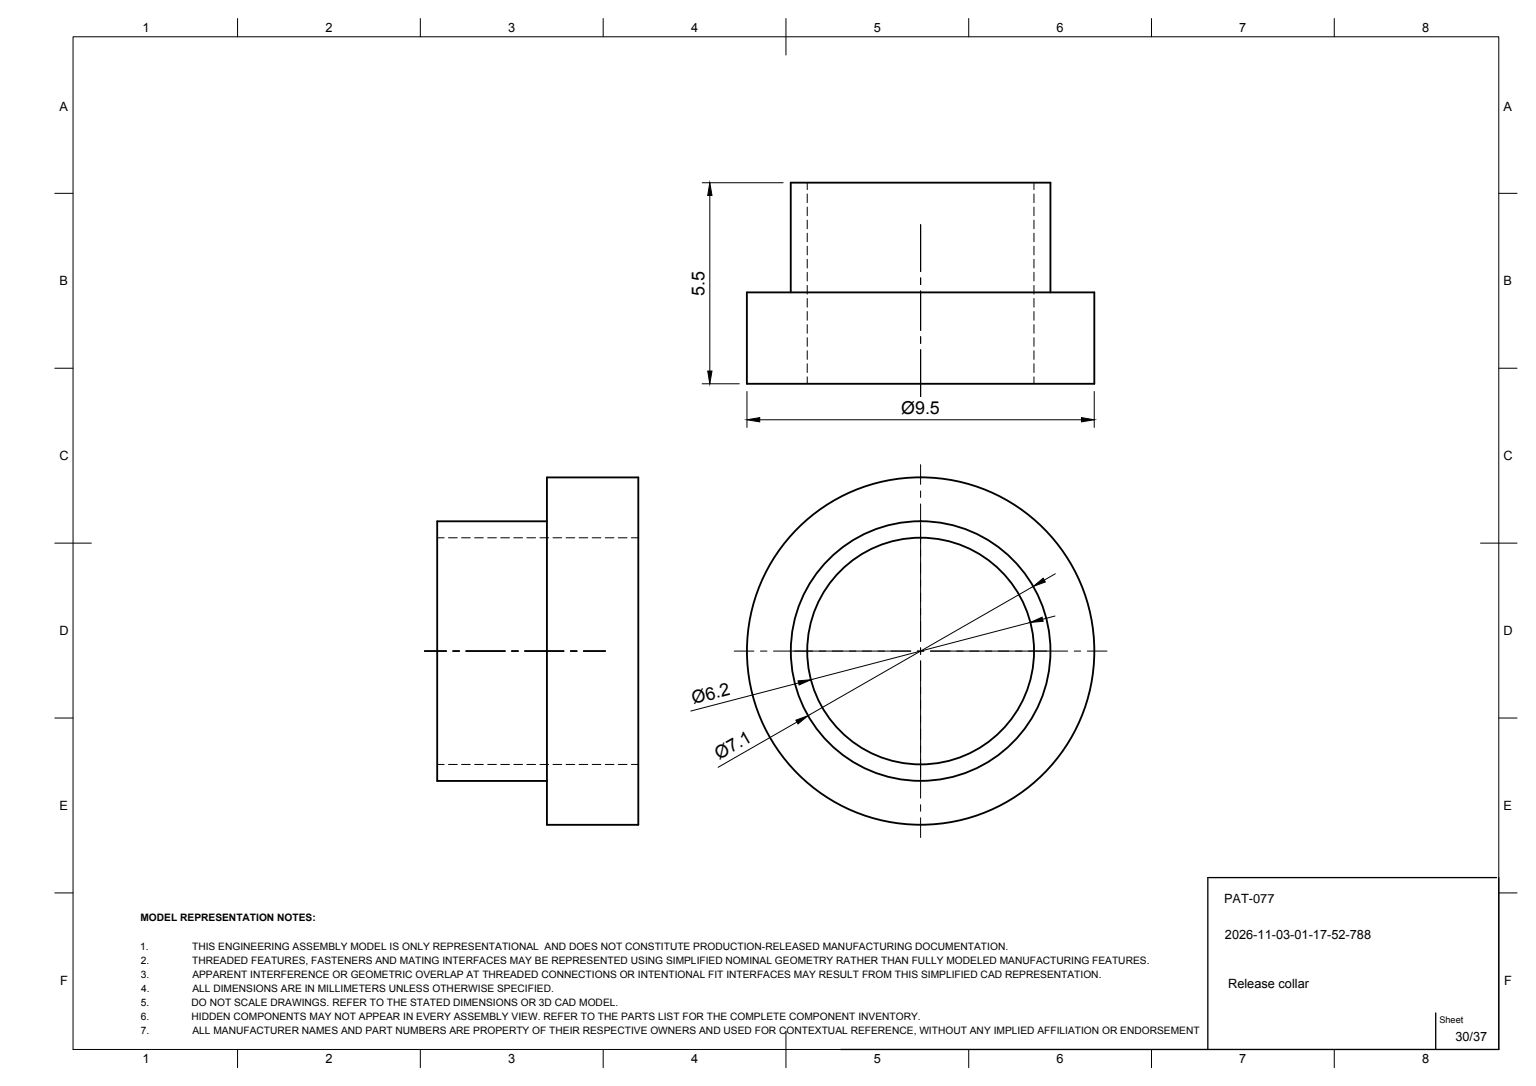
ISO-10303-21;
HEADER;
/* Generated by software containing ST-Developer
 * from STEP Tools, Inc. (www.steptools.com) 
 */

FILE_DESCRIPTION(
/* description */ ('Pallet stop with pneumatic fitting'),
/* implementation_level */ '2;1');

FILE_NAME(
/* name */ 'Release collar.step',
/* time_stamp */ '2026-10-27T10:51:41-07:00',
/* author */ (''),
/* organization */ (''),
/* preprocessor_version */ 'ST-DEVELOPER v20.2',
/* originating_system */ 'Autodesk Translation Framework v15.17.0.0',
/* authorisation */ '');

FILE_SCHEMA (('AUTOMOTIVE_DESIGN { 1 0 10303 214 3 1 1 }'));
ENDSEC;

DATA;
#10=MECHANICAL_DESIGN_GEOMETRIC_PRESENTATION_REPRESENTATION('',(#379),#10265);
#315=SHAPE_REPRESENTATION_RELATIONSHIP('SRR','None',#10430,#347);
#347=ADVANCED_BREP_SHAPE_REPRESENTATION('',(#410),#10254);
#379=STYLED_ITEM('',(#10669),#410);
#410=MANIFOLD_SOLID_BREP('Body1',#5068);
#522=FACE_BOUND('',#1371,.T.);
#523=FACE_BOUND('',#1374,.T.);
#524=FACE_BOUND('',#1377,.T.);
#672=PLANE('',#5859);
#673=PLANE('',#5864);
#674=PLANE('',#5868);
#953=FACE_OUTER_BOUND('',#1370,.T.);
#954=FACE_OUTER_BOUND('',#1372,.T.);
#955=FACE_OUTER_BOUND('',#1373,.T.);
#956=FACE_OUTER_BOUND('',#1375,.T.);
#957=FACE_OUTER_BOUND('',#1376,.T.);
#958=FACE_OUTER_BOUND('',#1378,.T.);
#1370=EDGE_LOOP('',(#4226));
#1371=EDGE_LOOP('',(#4227));
#1372=EDGE_LOOP('',(#4228,#4229,#4230,#4231));
#1373=EDGE_LOOP('',(#4232));
#1374=EDGE_LOOP('',(#4233));
#1375=EDGE_LOOP('',(#4234,#4235,#4236,#4237));
#1376=EDGE_LOOP('',(#4238));
#1377=EDGE_LOOP('',(#4239));
#1378=EDGE_LOOP('',(#4240,#4241,#4242,#4243));
#1709=LINE('',#9622,#2044);
#1710=LINE('',#9629,#2045);
#1711=LINE('',#9634,#2046);
#2044=VECTOR('',#7172,0.475);
#2045=VECTOR('',#7181,0.355);
#2046=VECTOR('',#7188,0.31);
#2342=CIRCLE('',#5860,0.475);
#2343=CIRCLE('',#5861,0.31);
#2344=CIRCLE('',#5863,0.475);
#2345=CIRCLE('',#5865,0.355);
#2346=CIRCLE('',#5867,0.355);
#2347=CIRCLE('',#5869,0.31);
#2676=VERTEX_POINT('',#9615);
#2677=VERTEX_POINT('',#9617);
#2678=VERTEX_POINT('',#9620);
#2679=VERTEX_POINT('',#9624);
#2680=VERTEX_POINT('',#9627);
#2681=VERTEX_POINT('',#9631);
#3212=EDGE_CURVE('',#2676,#2676,#2342,.T.);
#3213=EDGE_CURVE('',#2677,#2677,#2343,.T.);
#3214=EDGE_CURVE('',#2678,#2678,#2344,.T.);
#3215=EDGE_CURVE('',#2678,#2676,#1709,.T.);
#3216=EDGE_CURVE('',#2679,#2679,#2345,.T.);
#3217=EDGE_CURVE('',#2680,#2680,#2346,.T.);
#3218=EDGE_CURVE('',#2680,#2679,#1710,.T.);
#3219=EDGE_CURVE('',#2681,#2681,#2347,.T.);
#3220=EDGE_CURVE('',#2681,#2677,#1711,.T.);
#4226=ORIENTED_EDGE('',*,*,#3212,.F.);
#4227=ORIENTED_EDGE('',*,*,#3213,.T.);
#4228=ORIENTED_EDGE('',*,*,#3214,.F.);
#4229=ORIENTED_EDGE('',*,*,#3215,.T.);
#4230=ORIENTED_EDGE('',*,*,#3212,.T.);
#4231=ORIENTED_EDGE('',*,*,#3215,.F.);
#4232=ORIENTED_EDGE('',*,*,#3214,.T.);
#4233=ORIENTED_EDGE('',*,*,#3216,.F.);
#4234=ORIENTED_EDGE('',*,*,#3217,.F.);
#4235=ORIENTED_EDGE('',*,*,#3218,.T.);
#4236=ORIENTED_EDGE('',*,*,#3216,.T.);
#4237=ORIENTED_EDGE('',*,*,#3218,.F.);
#4238=ORIENTED_EDGE('',*,*,#3217,.T.);
#4239=ORIENTED_EDGE('',*,*,#3219,.F.);
#4240=ORIENTED_EDGE('',*,*,#3219,.T.);
#4241=ORIENTED_EDGE('',*,*,#3220,.T.);
#4242=ORIENTED_EDGE('',*,*,#3213,.F.);
#4243=ORIENTED_EDGE('',*,*,#3220,.F.);
#4707=CYLINDRICAL_SURFACE('',#5862,0.475);
#4708=CYLINDRICAL_SURFACE('',#5866,0.355);
#4709=CYLINDRICAL_SURFACE('',#5870,0.31);
#4948=ADVANCED_FACE('',(#953,#522),#672,.T.);
#4949=ADVANCED_FACE('',(#954),#4707,.T.);
#4950=ADVANCED_FACE('',(#955,#523),#673,.T.);
#4951=ADVANCED_FACE('',(#956),#4708,.T.);
#4952=ADVANCED_FACE('',(#957,#524),#674,.T.);
#4953=ADVANCED_FACE('',(#958),#4709,.F.);
#5068=CLOSED_SHELL('',(#4948,#4949,#4950,#4951,#4952,#4953));
#5858=AXIS2_PLACEMENT_3D('',#9613,#7160,#7161);
#5859=AXIS2_PLACEMENT_3D('',#9614,#7162,#7163);
#5860=AXIS2_PLACEMENT_3D('',#9616,#7164,#7165);
#5861=AXIS2_PLACEMENT_3D('',#9618,#7166,#7167);
#5862=AXIS2_PLACEMENT_3D('',#9619,#7168,#7169);
#5863=AXIS2_PLACEMENT_3D('',#9621,#7170,#7171);
#5864=AXIS2_PLACEMENT_3D('',#9623,#7173,#7174);
#5865=AXIS2_PLACEMENT_3D('',#9625,#7175,#7176);
#5866=AXIS2_PLACEMENT_3D('',#9626,#7177,#7178);
#5867=AXIS2_PLACEMENT_3D('',#9628,#7179,#7180);
#5868=AXIS2_PLACEMENT_3D('',#9630,#7182,#7183);
#5869=AXIS2_PLACEMENT_3D('',#9632,#7184,#7185);
#5870=AXIS2_PLACEMENT_3D('',#9633,#7186,#7187);
#7160=DIRECTION('axis',(0.,0.,1.));
#7161=DIRECTION('refdir',(1.,0.,0.));
#7162=DIRECTION('center_axis',(0.,1.,0.));
#7163=DIRECTION('ref_axis',(0.,0.,1.));
#7164=DIRECTION('center_axis',(0.,-1.,0.));
#7165=DIRECTION('ref_axis',(1.,0.,0.));
#7166=DIRECTION('center_axis',(0.,-1.,0.));
#7167=DIRECTION('ref_axis',(1.,0.,0.));
#7168=DIRECTION('center_axis',(0.,-1.,0.));
#7169=DIRECTION('ref_axis',(1.,0.,0.));
#7170=DIRECTION('center_axis',(0.,-1.,0.));
#7171=DIRECTION('ref_axis',(1.,0.,0.));
#7172=DIRECTION('',(0.,1.,0.));
#7173=DIRECTION('center_axis',(0.,-1.,0.));
#7174=DIRECTION('ref_axis',(0.,0.,-1.));
#7175=DIRECTION('center_axis',(0.,-1.,0.));
#7176=DIRECTION('ref_axis',(1.,0.,0.));
#7177=DIRECTION('center_axis',(0.,-1.,0.));
#7178=DIRECTION('ref_axis',(1.,0.,0.));
#7179=DIRECTION('center_axis',(0.,-1.,0.));
#7180=DIRECTION('ref_axis',(1.,0.,0.));
#7181=DIRECTION('',(0.,1.,0.));
#7182=DIRECTION('center_axis',(0.,-1.,0.));
#7183=DIRECTION('ref_axis',(0.,0.,-1.));
#7184=DIRECTION('center_axis',(0.,-1.,0.));
#7185=DIRECTION('ref_axis',(1.,0.,0.));
#7186=DIRECTION('center_axis',(0.,-1.,0.));
#7187=DIRECTION('ref_axis',(1.,0.,0.));
#7188=DIRECTION('',(0.,1.,0.));
#9613=CARTESIAN_POINT('',(0.,0.,0.));
#9614=CARTESIAN_POINT('Origin',(0.475,1.95,0.));
#9615=CARTESIAN_POINT('',(-0.475,1.95,-5.81707229594993E-17));
#9616=CARTESIAN_POINT('Origin',(0.,1.95,0.));
#9617=CARTESIAN_POINT('',(-0.31,1.95,-3.7964050773568E-17));
#9618=CARTESIAN_POINT('Origin',(0.,1.95,0.));
#9619=CARTESIAN_POINT('Origin',(0.,1.825,0.));
#9620=CARTESIAN_POINT('',(-0.475,1.7,-5.81707229594993E-17));
#9621=CARTESIAN_POINT('Origin',(0.,1.7,0.));
#9622=CARTESIAN_POINT('',(-0.475,1.825,-5.81707229594993E-17));
#9623=CARTESIAN_POINT('Origin',(0.355,1.7,0.));
#9624=CARTESIAN_POINT('',(-0.355,1.7,-4.3474961369731E-17));
#9625=CARTESIAN_POINT('Origin',(0.,1.7,0.));
#9626=CARTESIAN_POINT('Origin',(0.,1.55,0.));
#9627=CARTESIAN_POINT('',(-0.355,1.4,-4.3474961369731E-17));
#9628=CARTESIAN_POINT('Origin',(0.,1.4,0.));
#9629=CARTESIAN_POINT('',(-0.355,1.55,-4.3474961369731E-17));
#9630=CARTESIAN_POINT('Origin',(0.31,1.4,0.));
#9631=CARTESIAN_POINT('',(-0.31,1.4,-3.7964050773568E-17));
#9632=CARTESIAN_POINT('Origin',(0.,1.4,0.));
#9633=CARTESIAN_POINT('Origin',(0.,1.675,0.));
#9634=CARTESIAN_POINT('',(-0.31,1.675,-3.7964050773568E-17));
#10216=UNCERTAINTY_MEASURE_WITH_UNIT(LENGTH_MEASURE(0.001),#10266,
'DISTANCE_ACCURACY_VALUE',
'Maximum model space distance between geometric entities at asserted c
onnectivities');
#10227=UNCERTAINTY_MEASURE_WITH_UNIT(LENGTH_MEASURE(0.001),#10266,
'DISTANCE_ACCURACY_VALUE',
'Maximum model space distance between geometric entities at asserted c
onnectivities');
#10254=(
GEOMETRIC_REPRESENTATION_CONTEXT(3)
GLOBAL_UNCERTAINTY_ASSIGNED_CONTEXT((#10216))
GLOBAL_UNIT_ASSIGNED_CONTEXT((#10266,#10268,#10269))
REPRESENTATION_CONTEXT('','3D')
);
#10265=(
GEOMETRIC_REPRESENTATION_CONTEXT(3)
GLOBAL_UNCERTAINTY_ASSIGNED_CONTEXT((#10227))
GLOBAL_UNIT_ASSIGNED_CONTEXT((#10266,#10268,#10269))
REPRESENTATION_CONTEXT('','3D')
);
#10266=(
LENGTH_UNIT()
NAMED_UNIT(*)
SI_UNIT(.CENTI.,.METRE.)
);
#10268=(
NAMED_UNIT(*)
PLANE_ANGLE_UNIT()
SI_UNIT($,.RADIAN.)
);
#10269=(
NAMED_UNIT(*)
SI_UNIT($,.STERADIAN.)
SOLID_ANGLE_UNIT()
);
#10296=SHAPE_DEFINITION_REPRESENTATION(#10335,#10430);
#10335=PRODUCT_DEFINITION_SHAPE('',$,#10468);
#10430=SHAPE_REPRESENTATION('',(#5858),#10254);
#10441=PRODUCT_DEFINITION_CONTEXT('part definition',#10554,'design');
#10468=PRODUCT_DEFINITION('Release collar','Release collar',#10505,#10441);
#10505=PRODUCT_DEFINITION_FORMATION('',$,#10582);
#10554=APPLICATION_CONTEXT(
'Core Data for Automotive Mechanical Design Process');
#10555=PRODUCT_CONTEXT('part definition',#10554,'mechanical');
#10582=PRODUCT('Release collar','Release collar','Release collar',(#10555));
#10663=COLOUR_RGB('Off White',0.89,0.88,0.83);
#10664=FILL_AREA_STYLE_COLOUR('',#10663);
#10665=FILL_AREA_STYLE('',(#10664));
#10666=SURFACE_STYLE_FILL_AREA(#10665);
#10667=SURFACE_SIDE_STYLE('',(#10666));
#10668=SURFACE_STYLE_USAGE(.BOTH.,#10667);
#10669=PRESENTATION_STYLE_ASSIGNMENT((#10668));
ENDSEC;
END-ISO-10303-21;
